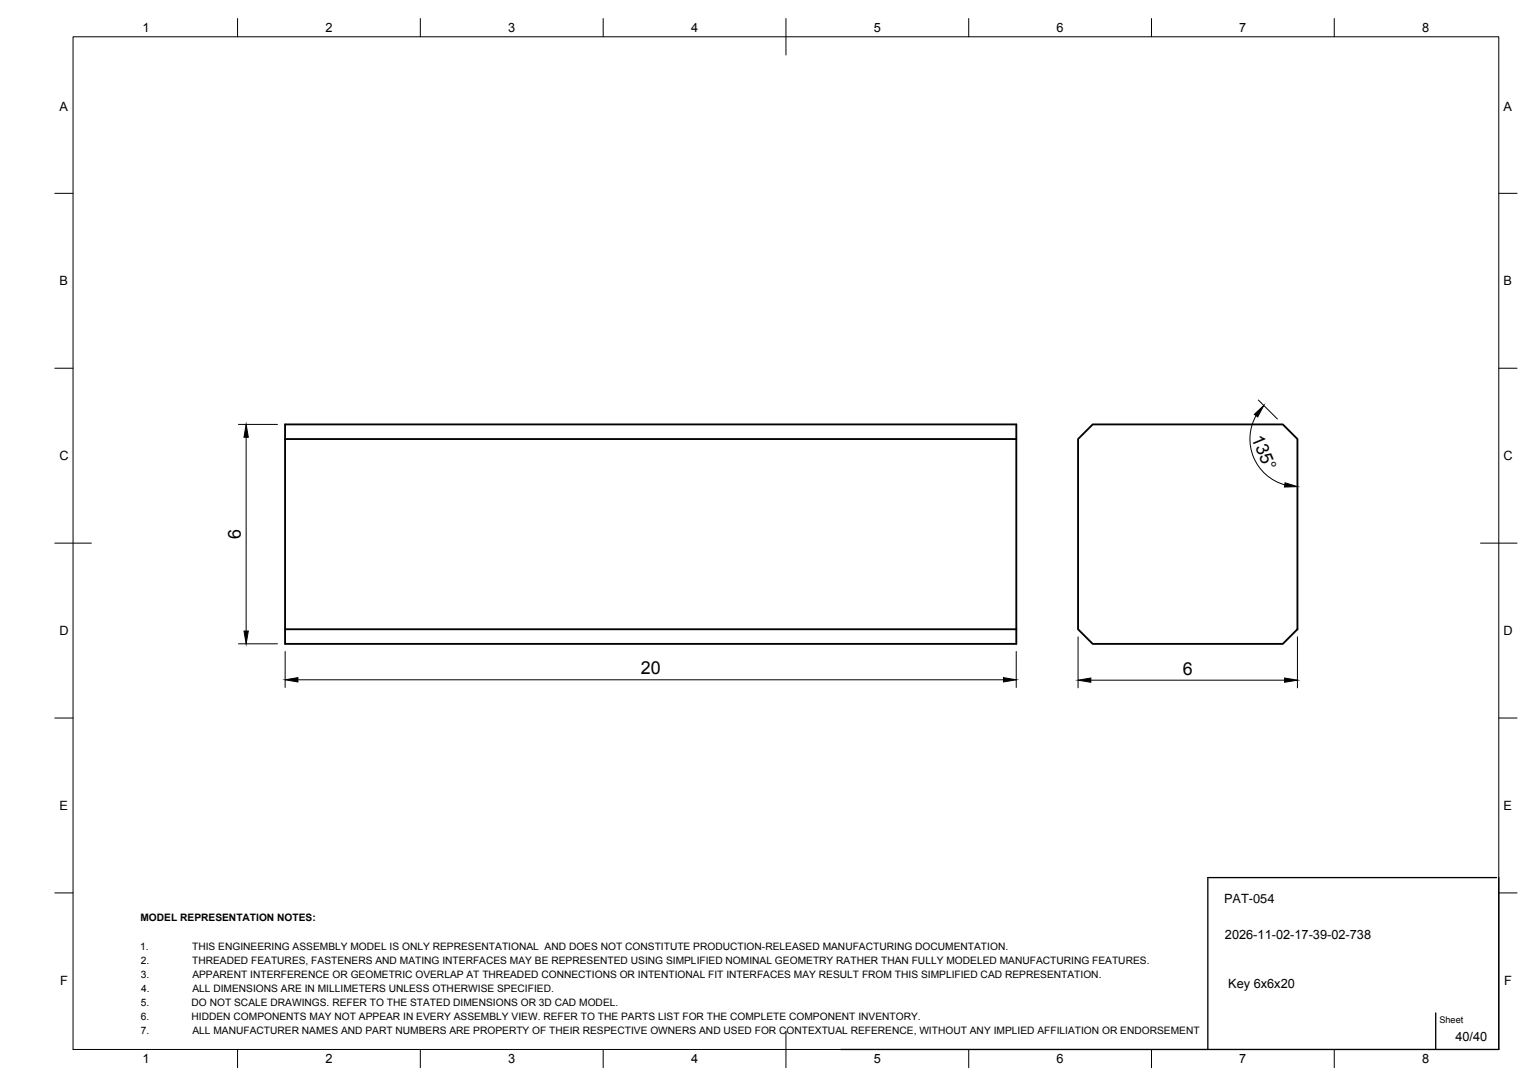
ISO-10303-21;
HEADER;
/* Generated by software containing ST-Developer
 * from STEP Tools, Inc. (www.steptools.com) 
 */

FILE_DESCRIPTION(
/* description */ ('PAT-054'),
/* implementation_level */ '2;1');

FILE_NAME(
/* name */ 'Key 6x6x20.step',
/* time_stamp */ '2026-10-29T16:38:13-07:00',
/* author */ (''),
/* organization */ (''),
/* preprocessor_version */ 'ST-DEVELOPER v20.2',
/* originating_system */ 'Autodesk Translation Framework v15.17.0.0',
/* authorisation */ '');

FILE_SCHEMA (('AUTOMOTIVE_DESIGN { 1 0 10303 214 3 1 1 }'));
ENDSEC;

DATA;
#10=MECHANICAL_DESIGN_GEOMETRIC_PRESENTATION_REPRESENTATION('',(#954),#33981);
#851=SHAPE_REPRESENTATION_RELATIONSHIP('SRR','None',#34229,#895);
#895=ADVANCED_BREP_SHAPE_REPRESENTATION('',(#1009),#33977);
#954=STYLED_ITEM('',(#34517),#1009);
#1009=MANIFOLD_SOLID_BREP('Body1',#13069);
#1543=PLANE('',#14767);
#1544=PLANE('',#14768);
#1545=PLANE('',#14769);
#1546=PLANE('',#14770);
#1547=PLANE('',#14771);
#1548=PLANE('',#14772);
#1549=PLANE('',#14773);
#1550=PLANE('',#14774);
#1551=PLANE('',#14775);
#1552=PLANE('',#14776);
#2255=FACE_OUTER_BOUND('',#3190,.T.);
#2256=FACE_OUTER_BOUND('',#3191,.T.);
#2257=FACE_OUTER_BOUND('',#3192,.T.);
#2258=FACE_OUTER_BOUND('',#3193,.T.);
#2259=FACE_OUTER_BOUND('',#3194,.T.);
#2260=FACE_OUTER_BOUND('',#3195,.T.);
#2261=FACE_OUTER_BOUND('',#3196,.T.);
#2262=FACE_OUTER_BOUND('',#3197,.T.);
#2263=FACE_OUTER_BOUND('',#3198,.T.);
#2264=FACE_OUTER_BOUND('',#3199,.T.);
#3190=EDGE_LOOP('',(#11805,#11806,#11807,#11808,#11809,#11810,#11811,#11812));
#3191=EDGE_LOOP('',(#11813,#11814,#11815,#11816));
#3192=EDGE_LOOP('',(#11817,#11818,#11819,#11820));
#3193=EDGE_LOOP('',(#11821,#11822,#11823,#11824));
#3194=EDGE_LOOP('',(#11825,#11826,#11827,#11828));
#3195=EDGE_LOOP('',(#11829,#11830,#11831,#11832,#11833,#11834,#11835,#11836));
#3196=EDGE_LOOP('',(#11837,#11838,#11839,#11840));
#3197=EDGE_LOOP('',(#11841,#11842,#11843,#11844));
#3198=EDGE_LOOP('',(#11845,#11846,#11847,#11848));
#3199=EDGE_LOOP('',(#11849,#11850,#11851,#11852));
#4100=LINE('',#33631,#5034);
#4101=LINE('',#33633,#5035);
#4102=LINE('',#33635,#5036);
#4103=LINE('',#33637,#5037);
#4104=LINE('',#33639,#5038);
#4105=LINE('',#33641,#5039);
#4106=LINE('',#33643,#5040);
#4107=LINE('',#33644,#5041);
#4108=LINE('',#33647,#5042);
#4109=LINE('',#33649,#5043);
#4110=LINE('',#33650,#5044);
#4111=LINE('',#33653,#5045);
#4112=LINE('',#33654,#5046);
#4113=LINE('',#33657,#5047);
#4114=LINE('',#33658,#5048);
#4115=LINE('',#33661,#5049);
#4116=LINE('',#33662,#5050);
#4117=LINE('',#33666,#5051);
#4118=LINE('',#33667,#5052);
#4119=LINE('',#33669,#5053);
#4120=LINE('',#33670,#5054);
#4121=LINE('',#33672,#5055);
#4122=LINE('',#33674,#5056);
#4123=LINE('',#33676,#5057);
#5034=VECTOR('',#18171,1.);
#5035=VECTOR('',#18172,1.);
#5036=VECTOR('',#18173,1.);
#5037=VECTOR('',#18174,1.);
#5038=VECTOR('',#18175,1.);
#5039=VECTOR('',#18176,1.);
#5040=VECTOR('',#18177,1.);
#5041=VECTOR('',#18178,1.);
#5042=VECTOR('',#18181,1.);
#5043=VECTOR('',#18182,1.);
#5044=VECTOR('',#18183,1.);
#5045=VECTOR('',#18186,1.);
#5046=VECTOR('',#18187,1.);
#5047=VECTOR('',#18190,1.);
#5048=VECTOR('',#18191,1.);
#5049=VECTOR('',#18194,1.);
#5050=VECTOR('',#18195,1.);
#5051=VECTOR('',#18198,1.);
#5052=VECTOR('',#18199,1.);
#5053=VECTOR('',#18200,1.);
#5054=VECTOR('',#18201,1.);
#5055=VECTOR('',#18204,1.);
#5056=VECTOR('',#18207,1.);
#5057=VECTOR('',#18210,1.);
#6688=VERTEX_POINT('',#33629);
#6689=VERTEX_POINT('',#33630);
#6690=VERTEX_POINT('',#33632);
#6691=VERTEX_POINT('',#33634);
#6692=VERTEX_POINT('',#33636);
#6693=VERTEX_POINT('',#33638);
#6694=VERTEX_POINT('',#33640);
#6695=VERTEX_POINT('',#33642);
#6696=VERTEX_POINT('',#33646);
#6697=VERTEX_POINT('',#33648);
#6698=VERTEX_POINT('',#33652);
#6699=VERTEX_POINT('',#33656);
#6700=VERTEX_POINT('',#33660);
#6701=VERTEX_POINT('',#33664);
#6702=VERTEX_POINT('',#33665);
#6703=VERTEX_POINT('',#33668);
#8402=EDGE_CURVE('',#6688,#6689,#4100,.T.);
#8403=EDGE_CURVE('',#6690,#6688,#4101,.T.);
#8404=EDGE_CURVE('',#6691,#6690,#4102,.T.);
#8405=EDGE_CURVE('',#6692,#6691,#4103,.T.);
#8406=EDGE_CURVE('',#6693,#6692,#4104,.T.);
#8407=EDGE_CURVE('',#6694,#6693,#4105,.T.);
#8408=EDGE_CURVE('',#6695,#6694,#4106,.T.);
#8409=EDGE_CURVE('',#6689,#6695,#4107,.T.);
#8410=EDGE_CURVE('',#6692,#6696,#4108,.T.);
#8411=EDGE_CURVE('',#6696,#6697,#4109,.T.);
#8412=EDGE_CURVE('',#6697,#6693,#4110,.T.);
#8413=EDGE_CURVE('',#6698,#6691,#4111,.T.);
#8414=EDGE_CURVE('',#6698,#6696,#4112,.T.);
#8415=EDGE_CURVE('',#6690,#6699,#4113,.T.);
#8416=EDGE_CURVE('',#6699,#6698,#4114,.T.);
#8417=EDGE_CURVE('',#6700,#6688,#4115,.T.);
#8418=EDGE_CURVE('',#6700,#6699,#4116,.T.);
#8419=EDGE_CURVE('',#6701,#6702,#4117,.T.);
#8420=EDGE_CURVE('',#6697,#6701,#4118,.T.);
#8421=EDGE_CURVE('',#6703,#6700,#4119,.T.);
#8422=EDGE_CURVE('',#6702,#6703,#4120,.T.);
#8423=EDGE_CURVE('',#6694,#6701,#4121,.T.);
#8424=EDGE_CURVE('',#6689,#6703,#4122,.T.);
#8425=EDGE_CURVE('',#6702,#6695,#4123,.T.);
#11805=ORIENTED_EDGE('',*,*,#8402,.F.);
#11806=ORIENTED_EDGE('',*,*,#8403,.F.);
#11807=ORIENTED_EDGE('',*,*,#8404,.F.);
#11808=ORIENTED_EDGE('',*,*,#8405,.F.);
#11809=ORIENTED_EDGE('',*,*,#8406,.F.);
#11810=ORIENTED_EDGE('',*,*,#8407,.F.);
#11811=ORIENTED_EDGE('',*,*,#8408,.F.);
#11812=ORIENTED_EDGE('',*,*,#8409,.F.);
#11813=ORIENTED_EDGE('',*,*,#8406,.T.);
#11814=ORIENTED_EDGE('',*,*,#8410,.T.);
#11815=ORIENTED_EDGE('',*,*,#8411,.T.);
#11816=ORIENTED_EDGE('',*,*,#8412,.T.);
#11817=ORIENTED_EDGE('',*,*,#8405,.T.);
#11818=ORIENTED_EDGE('',*,*,#8413,.F.);
#11819=ORIENTED_EDGE('',*,*,#8414,.T.);
#11820=ORIENTED_EDGE('',*,*,#8410,.F.);
#11821=ORIENTED_EDGE('',*,*,#8404,.T.);
#11822=ORIENTED_EDGE('',*,*,#8415,.T.);
#11823=ORIENTED_EDGE('',*,*,#8416,.T.);
#11824=ORIENTED_EDGE('',*,*,#8413,.T.);
#11825=ORIENTED_EDGE('',*,*,#8403,.T.);
#11826=ORIENTED_EDGE('',*,*,#8417,.F.);
#11827=ORIENTED_EDGE('',*,*,#8418,.T.);
#11828=ORIENTED_EDGE('',*,*,#8415,.F.);
#11829=ORIENTED_EDGE('',*,*,#8419,.F.);
#11830=ORIENTED_EDGE('',*,*,#8420,.F.);
#11831=ORIENTED_EDGE('',*,*,#8411,.F.);
#11832=ORIENTED_EDGE('',*,*,#8414,.F.);
#11833=ORIENTED_EDGE('',*,*,#8416,.F.);
#11834=ORIENTED_EDGE('',*,*,#8418,.F.);
#11835=ORIENTED_EDGE('',*,*,#8421,.F.);
#11836=ORIENTED_EDGE('',*,*,#8422,.F.);
#11837=ORIENTED_EDGE('',*,*,#8407,.T.);
#11838=ORIENTED_EDGE('',*,*,#8412,.F.);
#11839=ORIENTED_EDGE('',*,*,#8420,.T.);
#11840=ORIENTED_EDGE('',*,*,#8423,.F.);
#11841=ORIENTED_EDGE('',*,*,#8402,.T.);
#11842=ORIENTED_EDGE('',*,*,#8424,.T.);
#11843=ORIENTED_EDGE('',*,*,#8421,.T.);
#11844=ORIENTED_EDGE('',*,*,#8417,.T.);
#11845=ORIENTED_EDGE('',*,*,#8408,.T.);
#11846=ORIENTED_EDGE('',*,*,#8423,.T.);
#11847=ORIENTED_EDGE('',*,*,#8419,.T.);
#11848=ORIENTED_EDGE('',*,*,#8425,.T.);
#11849=ORIENTED_EDGE('',*,*,#8409,.T.);
#11850=ORIENTED_EDGE('',*,*,#8425,.F.);
#11851=ORIENTED_EDGE('',*,*,#8422,.T.);
#11852=ORIENTED_EDGE('',*,*,#8424,.F.);
#12967=ADVANCED_FACE('',(#2255),#1543,.F.);
#12968=ADVANCED_FACE('',(#2256),#1544,.T.);
#12969=ADVANCED_FACE('',(#2257),#1545,.T.);
#12970=ADVANCED_FACE('',(#2258),#1546,.T.);
#12971=ADVANCED_FACE('',(#2259),#1547,.T.);
#12972=ADVANCED_FACE('',(#2260),#1548,.T.);
#12973=ADVANCED_FACE('',(#2261),#1549,.F.);
#12974=ADVANCED_FACE('',(#2262),#1550,.T.);
#12975=ADVANCED_FACE('',(#2263),#1551,.T.);
#12976=ADVANCED_FACE('',(#2264),#1552,.T.);
#13069=CLOSED_SHELL('',(#12967,#12968,#12969,#12970,#12971,#12972,#12973,
#12974,#12975,#12976));
#14766=AXIS2_PLACEMENT_3D('',#33627,#18167,#18168);
#14767=AXIS2_PLACEMENT_3D('',#33628,#18169,#18170);
#14768=AXIS2_PLACEMENT_3D('',#33645,#18179,#18180);
#14769=AXIS2_PLACEMENT_3D('',#33651,#18184,#18185);
#14770=AXIS2_PLACEMENT_3D('',#33655,#18188,#18189);
#14771=AXIS2_PLACEMENT_3D('',#33659,#18192,#18193);
#14772=AXIS2_PLACEMENT_3D('',#33663,#18196,#18197);
#14773=AXIS2_PLACEMENT_3D('',#33671,#18202,#18203);
#14774=AXIS2_PLACEMENT_3D('',#33673,#18205,#18206);
#14775=AXIS2_PLACEMENT_3D('',#33675,#18208,#18209);
#14776=AXIS2_PLACEMENT_3D('',#33677,#18211,#18212);
#18167=DIRECTION('axis',(0.,0.,1.));
#18168=DIRECTION('refdir',(1.,0.,0.));
#18169=DIRECTION('center_axis',(1.,0.,0.));
#18170=DIRECTION('ref_axis',(0.,0.,-1.));
#18171=DIRECTION('',(0.,-0.707106781186547,-0.707106781186548));
#18172=DIRECTION('',(0.,-1.,0.));
#18173=DIRECTION('',(0.,-0.707106781186547,0.707106781186548));
#18174=DIRECTION('',(0.,0.,1.));
#18175=DIRECTION('',(0.,0.707106781186547,0.707106781186548));
#18176=DIRECTION('',(0.,1.,0.));
#18177=DIRECTION('',(0.,0.707106781186547,-0.707106781186548));
#18178=DIRECTION('',(0.,0.,-1.));
#18179=DIRECTION('center_axis',(0.,0.707106781186548,-0.707106781186547));
#18180=DIRECTION('ref_axis',(-1.,0.,0.));
#18181=DIRECTION('',(1.,0.,0.));
#18182=DIRECTION('',(0.,-0.707106781186547,-0.707106781186548));
#18183=DIRECTION('',(-1.,0.,0.));
#18184=DIRECTION('center_axis',(0.,1.,0.));
#18185=DIRECTION('ref_axis',(-1.,0.,0.));
#18186=DIRECTION('',(-1.,0.,0.));
#18187=DIRECTION('',(0.,0.,-1.));
#18188=DIRECTION('center_axis',(0.,0.707106781186548,0.707106781186547));
#18189=DIRECTION('ref_axis',(1.,0.,0.));
#18190=DIRECTION('',(1.,0.,0.));
#18191=DIRECTION('',(0.,0.707106781186547,-0.707106781186548));
#18192=DIRECTION('center_axis',(0.,0.,1.));
#18193=DIRECTION('ref_axis',(1.,0.,0.));
#18194=DIRECTION('',(-1.,0.,0.));
#18195=DIRECTION('',(0.,1.,0.));
#18196=DIRECTION('center_axis',(1.,0.,0.));
#18197=DIRECTION('ref_axis',(0.,0.,-1.));
#18198=DIRECTION('',(0.,-0.707106781186547,0.707106781186548));
#18199=DIRECTION('',(0.,-1.,0.));
#18200=DIRECTION('',(0.,0.707106781186547,0.707106781186548));
#18201=DIRECTION('',(0.,0.,1.));
#18202=DIRECTION('center_axis',(0.,0.,1.));
#18203=DIRECTION('ref_axis',(1.,0.,0.));
#18204=DIRECTION('',(1.,0.,0.));
#18205=DIRECTION('center_axis',(0.,-0.707106781186548,0.707106781186547));
#18206=DIRECTION('ref_axis',(1.,0.,0.));
#18207=DIRECTION('',(1.,0.,0.));
#18208=DIRECTION('center_axis',(0.,-0.707106781186548,-0.707106781186547));
#18209=DIRECTION('ref_axis',(-1.,0.,0.));
#18210=DIRECTION('',(-1.,0.,0.));
#18211=DIRECTION('center_axis',(0.,-1.,0.));
#18212=DIRECTION('ref_axis',(1.,0.,0.));
#33627=CARTESIAN_POINT('',(0.,0.,0.));
#33628=CARTESIAN_POINT('Origin',(-1.,0.,0.35));
#33629=CARTESIAN_POINT('',(-1.,-0.26,0.6));
#33630=CARTESIAN_POINT('',(-1.,-0.3,0.56));
#33631=CARTESIAN_POINT('',(-1.,-0.2675,0.5925));
#33632=CARTESIAN_POINT('',(-1.,0.26,0.6));
#33633=CARTESIAN_POINT('',(-1.,0.,0.6));
#33634=CARTESIAN_POINT('',(-1.,0.3,0.56));
#33635=CARTESIAN_POINT('',(-1.,0.2675,0.5925));
#33636=CARTESIAN_POINT('',(-1.,0.3,0.04));
#33637=CARTESIAN_POINT('',(-1.,0.3,0.175));
#33638=CARTESIAN_POINT('',(-1.,0.26,0.));
#33639=CARTESIAN_POINT('',(-1.,0.2925,0.0325));
#33640=CARTESIAN_POINT('',(-1.,-0.26,0.));
#33641=CARTESIAN_POINT('',(-1.,0.,0.));
#33642=CARTESIAN_POINT('',(-1.,-0.3,0.04));
#33643=CARTESIAN_POINT('',(-1.,-0.2925,0.0325));
#33644=CARTESIAN_POINT('',(-1.,-0.3,0.175));
#33645=CARTESIAN_POINT('Origin',(0.75,0.28,0.02));
#33646=CARTESIAN_POINT('',(1.,0.3,0.04));
#33647=CARTESIAN_POINT('',(0.75,0.3,0.04));
#33648=CARTESIAN_POINT('',(1.,0.26,0.));
#33649=CARTESIAN_POINT('',(1.,0.2925,0.0325));
#33650=CARTESIAN_POINT('',(0.75,0.26,0.));
#33651=CARTESIAN_POINT('Origin',(1.5,0.3,0.));
#33652=CARTESIAN_POINT('',(1.,0.3,0.56));
#33653=CARTESIAN_POINT('',(0.75,0.3,0.56));
#33654=CARTESIAN_POINT('',(1.,0.3,0.175));
#33655=CARTESIAN_POINT('Origin',(0.75,0.28,0.58));
#33656=CARTESIAN_POINT('',(1.,0.26,0.6));
#33657=CARTESIAN_POINT('',(0.75,0.26,0.6));
#33658=CARTESIAN_POINT('',(1.,0.2675,0.5925));
#33659=CARTESIAN_POINT('Origin',(0.,0.,0.6));
#33660=CARTESIAN_POINT('',(1.,-0.26,0.6));
#33661=CARTESIAN_POINT('',(-0.75,-0.26,0.6));
#33662=CARTESIAN_POINT('',(1.,0.,0.6));
#33663=CARTESIAN_POINT('Origin',(1.,0.,0.35));
#33664=CARTESIAN_POINT('',(1.,-0.26,0.));
#33665=CARTESIAN_POINT('',(1.,-0.3,0.04));
#33666=CARTESIAN_POINT('',(1.,-0.2925,0.0325));
#33667=CARTESIAN_POINT('',(1.,0.,0.));
#33668=CARTESIAN_POINT('',(1.,-0.3,0.56));
#33669=CARTESIAN_POINT('',(1.,-0.2675,0.5925));
#33670=CARTESIAN_POINT('',(1.,-0.3,0.175));
#33671=CARTESIAN_POINT('Origin',(0.,0.,0.));
#33672=CARTESIAN_POINT('',(-0.75,-0.26,0.));
#33673=CARTESIAN_POINT('Origin',(-0.75,-0.28,0.58));
#33674=CARTESIAN_POINT('',(-0.75,-0.3,0.56));
#33675=CARTESIAN_POINT('Origin',(-0.75,-0.28,0.02));
#33676=CARTESIAN_POINT('',(-0.75,-0.3,0.04));
#33677=CARTESIAN_POINT('Origin',(-1.5,-0.3,0.));
#33925=UNCERTAINTY_MEASURE_WITH_UNIT(LENGTH_MEASURE(0.001),#33982,
'DISTANCE_ACCURACY_VALUE',
'Maximum model space distance between geometric entities at asserted c
onnectivities');
#33929=UNCERTAINTY_MEASURE_WITH_UNIT(LENGTH_MEASURE(0.001),#33982,
'DISTANCE_ACCURACY_VALUE',
'Maximum model space distance between geometric entities at asserted c
onnectivities');
#33977=(
GEOMETRIC_REPRESENTATION_CONTEXT(3)
GLOBAL_UNCERTAINTY_ASSIGNED_CONTEXT((#33925))
GLOBAL_UNIT_ASSIGNED_CONTEXT((#33982,#33984,#33985))
REPRESENTATION_CONTEXT('','3D')
);
#33981=(
GEOMETRIC_REPRESENTATION_CONTEXT(3)
GLOBAL_UNCERTAINTY_ASSIGNED_CONTEXT((#33929))
GLOBAL_UNIT_ASSIGNED_CONTEXT((#33982,#33984,#33985))
REPRESENTATION_CONTEXT('','3D')
);
#33982=(
LENGTH_UNIT()
NAMED_UNIT(*)
SI_UNIT(.CENTI.,.METRE.)
);
#33984=(
NAMED_UNIT(*)
PLANE_ANGLE_UNIT()
SI_UNIT($,.RADIAN.)
);
#33985=(
NAMED_UNIT(*)
SI_UNIT($,.STERADIAN.)
SOLID_ANGLE_UNIT()
);
#34033=SHAPE_DEFINITION_REPRESENTATION(#34117,#34229);
#34117=PRODUCT_DEFINITION_SHAPE('',$,#34281);
#34229=SHAPE_REPRESENTATION('',(#14766),#33977);
#34233=PRODUCT_DEFINITION_CONTEXT('part definition',#34388,'design');
#34281=PRODUCT_DEFINITION('Key 6x6x20','Key 6x6x20',#34332,#34233);
#34332=PRODUCT_DEFINITION_FORMATION('',$,#34437);
#34388=APPLICATION_CONTEXT(
'Core Data for Automotive Mechanical Design Process');
#34389=PRODUCT_CONTEXT('part definition',#34388,'mechanical');
#34437=PRODUCT('Key 6x6x20','Key 6x6x20','Key 6x6x20',(#34389));
#34511=COLOUR_RGB('Grey',0.48,0.52,0.57);
#34512=FILL_AREA_STYLE_COLOUR('',#34511);
#34513=FILL_AREA_STYLE('',(#34512));
#34514=SURFACE_STYLE_FILL_AREA(#34513);
#34515=SURFACE_SIDE_STYLE('',(#34514));
#34516=SURFACE_STYLE_USAGE(.BOTH.,#34515);
#34517=PRESENTATION_STYLE_ASSIGNMENT((#34516));
ENDSEC;
END-ISO-10303-21;
